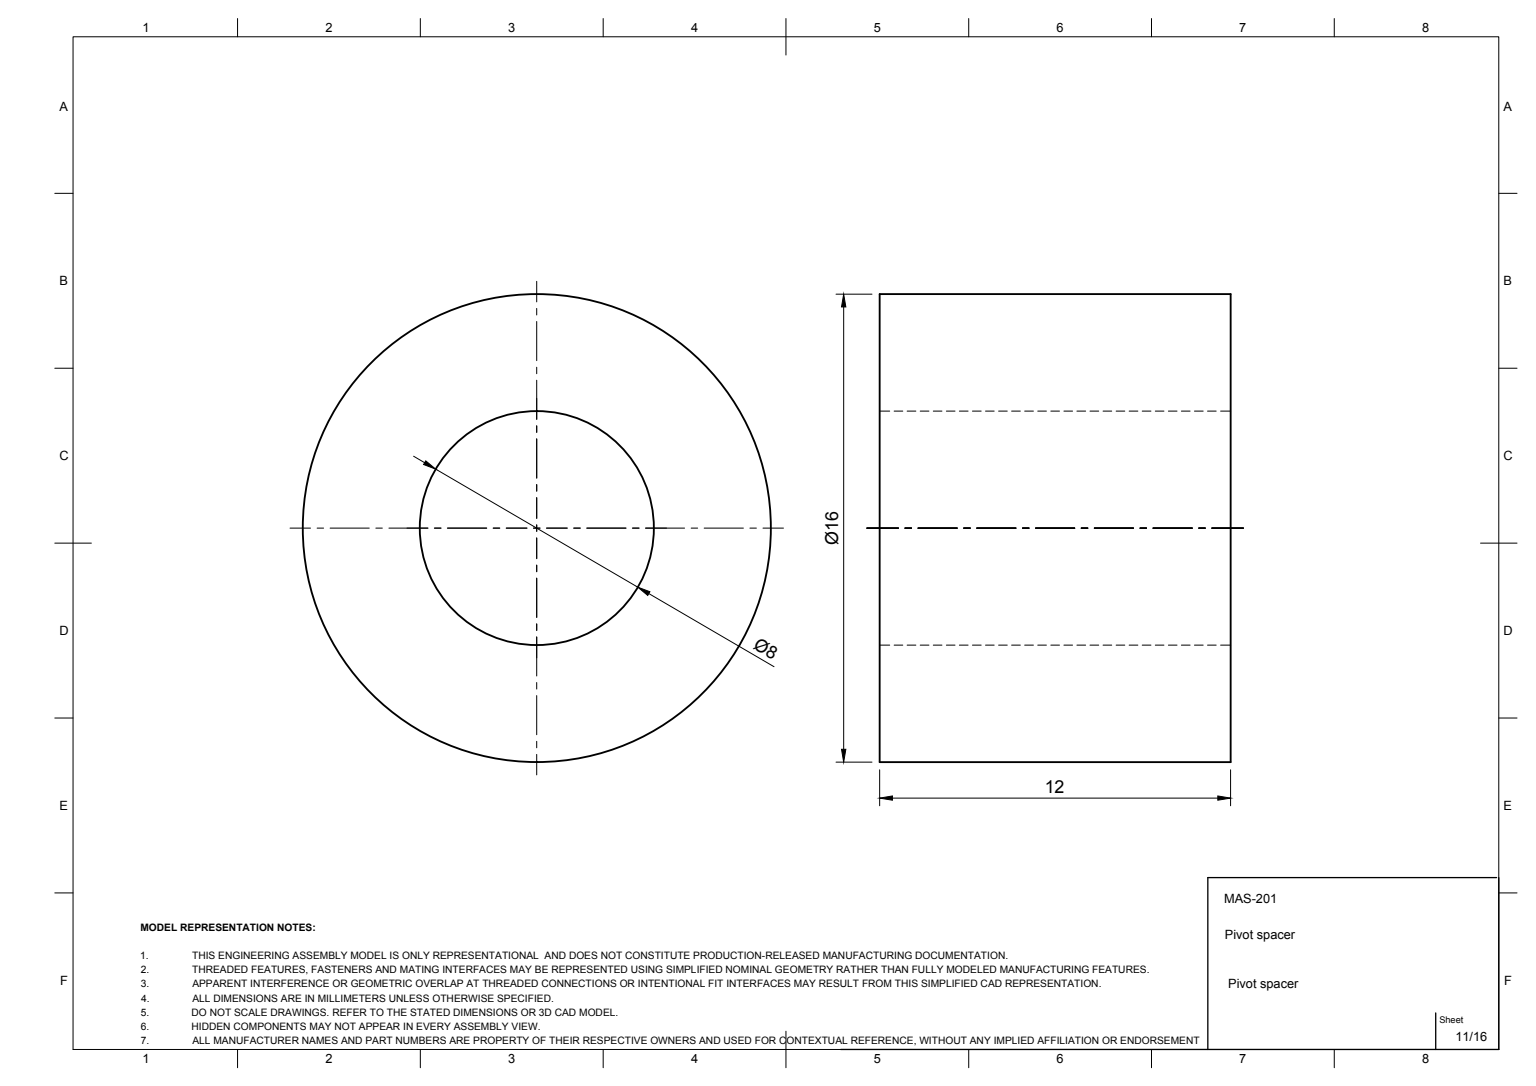
ISO-10303-21;
HEADER;
/* Generated by software containing ST-Developer
 * from STEP Tools, Inc. (www.steptools.com) 
 */

FILE_DESCRIPTION(
/* description */ ('Independent manual two-gate roller-track escapement for nominal30mm d
iameter20mm wide feed rollers. Opposed gates are driven by native capt
ured pin-slot loops with positive curved-slot travel stops at\X\B116de
g. Repeated gate/pin/washer/clip instances, adapted native common bear
ing families, full retaining lips and rotating polymer grip. External 
workpieces, gravity feeder/incline and mount anchors outside assembly.
 No powered-feed compatibility, impact, capacity, safety, force, wear 
or life rating.'),
/* implementation_level */ '2;1');

FILE_NAME(
/* name */ 'Pivot spacer.step',
/* time_stamp */ '2026-11-08T18:43:23-08:00',
/* author */ (''),
/* organization */ (''),
/* preprocessor_version */ 'ST-DEVELOPER v20.2',
/* originating_system */ 'Autodesk Translation Framework v15.17.0.0',
/* authorisation */ '');

FILE_SCHEMA (('AUTOMOTIVE_DESIGN { 1 0 10303 214 3 1 1 }'));
ENDSEC;

DATA;
#10=MECHANICAL_DESIGN_GEOMETRIC_PRESENTATION_REPRESENTATION('',(#465),#19863);
#427=SHAPE_REPRESENTATION_RELATIONSHIP('SRR','None',#19945,#446);
#446=ADVANCED_BREP_SHAPE_REPRESENTATION('',(#484),#19854);
#465=STYLED_ITEM('',(#20042),#484);
#484=MANIFOLD_SOLID_BREP('Body1',#6434);
#848=LINE('',#15905,#1313);
#849=LINE('',#15911,#1314);
#1313=VECTOR('',#8246,4.);
#1314=VECTOR('',#8253,8.);
#1552=CYLINDRICAL_SURFACE('',#7001,4.);
#1553=CYLINDRICAL_SURFACE('',#7004,8.);
#1671=FACE_BOUND('',#2349,.T.);
#1672=FACE_BOUND('',#2351,.T.);
#1933=FACE_OUTER_BOUND('',#2346,.T.);
#1934=FACE_OUTER_BOUND('',#2347,.T.);
#1935=FACE_OUTER_BOUND('',#2348,.T.);
#1936=FACE_OUTER_BOUND('',#2350,.T.);
#2346=EDGE_LOOP('',(#5397,#5398,#5399,#5400));
#2347=EDGE_LOOP('',(#5401,#5402,#5403,#5404));
#2348=EDGE_LOOP('',(#5405));
#2349=EDGE_LOOP('',(#5406));
#2350=EDGE_LOOP('',(#5407));
#2351=EDGE_LOOP('',(#5408));
#2570=CIRCLE('',#7002,4.);
#2571=CIRCLE('',#7003,4.);
#2572=CIRCLE('',#7005,8.);
#2573=CIRCLE('',#7006,8.);
#3044=VERTEX_POINT('',#15902);
#3045=VERTEX_POINT('',#15904);
#3046=VERTEX_POINT('',#15908);
#3047=VERTEX_POINT('',#15910);
#3857=EDGE_CURVE('',#3044,#3044,#2570,.T.);
#3858=EDGE_CURVE('',#3044,#3045,#848,.T.);
#3859=EDGE_CURVE('',#3045,#3045,#2571,.T.);
#3860=EDGE_CURVE('',#3046,#3046,#2572,.T.);
#3861=EDGE_CURVE('',#3046,#3047,#849,.T.);
#3862=EDGE_CURVE('',#3047,#3047,#2573,.T.);
#5397=ORIENTED_EDGE('',*,*,#3857,.F.);
#5398=ORIENTED_EDGE('',*,*,#3858,.T.);
#5399=ORIENTED_EDGE('',*,*,#3859,.T.);
#5400=ORIENTED_EDGE('',*,*,#3858,.F.);
#5401=ORIENTED_EDGE('',*,*,#3860,.F.);
#5402=ORIENTED_EDGE('',*,*,#3861,.T.);
#5403=ORIENTED_EDGE('',*,*,#3862,.T.);
#5404=ORIENTED_EDGE('',*,*,#3861,.F.);
#5405=ORIENTED_EDGE('',*,*,#3860,.T.);
#5406=ORIENTED_EDGE('',*,*,#3857,.T.);
#5407=ORIENTED_EDGE('',*,*,#3862,.F.);
#5408=ORIENTED_EDGE('',*,*,#3859,.F.);
#6024=PLANE('',#7007);
#6025=PLANE('',#7008);
#6312=ADVANCED_FACE('',(#1933),#1552,.F.);
#6313=ADVANCED_FACE('',(#1934),#1553,.T.);
#6314=ADVANCED_FACE('',(#1935,#1671),#6024,.T.);
#6315=ADVANCED_FACE('',(#1936,#1672),#6025,.F.);
#6434=CLOSED_SHELL('',(#6312,#6313,#6314,#6315));
#7000=AXIS2_PLACEMENT_3D('',#15900,#8240,#8241);
#7001=AXIS2_PLACEMENT_3D('',#15901,#8242,#8243);
#7002=AXIS2_PLACEMENT_3D('',#15903,#8244,#8245);
#7003=AXIS2_PLACEMENT_3D('',#15906,#8247,#8248);
#7004=AXIS2_PLACEMENT_3D('',#15907,#8249,#8250);
#7005=AXIS2_PLACEMENT_3D('',#15909,#8251,#8252);
#7006=AXIS2_PLACEMENT_3D('',#15912,#8254,#8255);
#7007=AXIS2_PLACEMENT_3D('',#15913,#8256,#8257);
#7008=AXIS2_PLACEMENT_3D('',#15914,#8258,#8259);
#8240=DIRECTION('axis',(0.,0.,1.));
#8241=DIRECTION('refdir',(1.,0.,0.));
#8242=DIRECTION('center_axis',(0.,0.,1.));
#8243=DIRECTION('ref_axis',(1.,0.,0.));
#8244=DIRECTION('center_axis',(0.,0.,-1.));
#8245=DIRECTION('ref_axis',(1.,0.,0.));
#8246=DIRECTION('',(0.,0.,-1.));
#8247=DIRECTION('center_axis',(0.,0.,-1.));
#8248=DIRECTION('ref_axis',(1.,0.,0.));
#8249=DIRECTION('center_axis',(0.,0.,1.));
#8250=DIRECTION('ref_axis',(1.,0.,0.));
#8251=DIRECTION('center_axis',(0.,0.,1.));
#8252=DIRECTION('ref_axis',(1.,0.,0.));
#8253=DIRECTION('',(0.,0.,-1.));
#8254=DIRECTION('center_axis',(0.,0.,1.));
#8255=DIRECTION('ref_axis',(1.,0.,0.));
#8256=DIRECTION('center_axis',(0.,0.,1.));
#8257=DIRECTION('ref_axis',(1.,0.,0.));
#8258=DIRECTION('center_axis',(0.,0.,1.));
#8259=DIRECTION('ref_axis',(1.,0.,0.));
#15900=CARTESIAN_POINT('',(0.,0.,0.));
#15901=CARTESIAN_POINT('Origin',(0.,0.,0.));
#15902=CARTESIAN_POINT('',(-4.,-4.89858719658941E-16,12.));
#15903=CARTESIAN_POINT('Origin',(0.,0.,12.));
#15904=CARTESIAN_POINT('',(-4.,-4.89858719658941E-16,0.));
#15905=CARTESIAN_POINT('',(-4.,-4.89858719658941E-16,0.));
#15906=CARTESIAN_POINT('Origin',(0.,0.,0.));
#15907=CARTESIAN_POINT('Origin',(0.,0.,0.));
#15908=CARTESIAN_POINT('',(-8.,-9.79717439317883E-16,12.));
#15909=CARTESIAN_POINT('Origin',(0.,0.,12.));
#15910=CARTESIAN_POINT('',(-8.,-9.79717439317883E-16,0.));
#15911=CARTESIAN_POINT('',(-8.,-9.79717439317883E-16,0.));
#15912=CARTESIAN_POINT('Origin',(0.,0.,0.));
#15913=CARTESIAN_POINT('Origin',(0.,0.,12.));
#15914=CARTESIAN_POINT('Origin',(0.,0.,0.));
#19833=UNCERTAINTY_MEASURE_WITH_UNIT(LENGTH_MEASURE(0.01),#19864,
'DISTANCE_ACCURACY_VALUE',
'Maximum model space distance between geometric entities at asserted c
onnectivities');
#19842=UNCERTAINTY_MEASURE_WITH_UNIT(LENGTH_MEASURE(0.01),#19864,
'DISTANCE_ACCURACY_VALUE',
'Maximum model space distance between geometric entities at asserted c
onnectivities');
#19854=(
GEOMETRIC_REPRESENTATION_CONTEXT(3)
GLOBAL_UNCERTAINTY_ASSIGNED_CONTEXT((#19833))
GLOBAL_UNIT_ASSIGNED_CONTEXT((#19864,#19866,#19867))
REPRESENTATION_CONTEXT('','3D')
);
#19863=(
GEOMETRIC_REPRESENTATION_CONTEXT(3)
GLOBAL_UNCERTAINTY_ASSIGNED_CONTEXT((#19842))
GLOBAL_UNIT_ASSIGNED_CONTEXT((#19864,#19866,#19867))
REPRESENTATION_CONTEXT('','3D')
);
#19864=(
LENGTH_UNIT()
NAMED_UNIT(*)
SI_UNIT(.MILLI.,.METRE.)
);
#19866=(
NAMED_UNIT(*)
PLANE_ANGLE_UNIT()
SI_UNIT($,.RADIAN.)
);
#19867=(
NAMED_UNIT(*)
SI_UNIT($,.STERADIAN.)
SOLID_ANGLE_UNIT()
);
#19879=SHAPE_DEFINITION_REPRESENTATION(#19899,#19945);
#19899=PRODUCT_DEFINITION_SHAPE('',$,#19966);
#19945=SHAPE_REPRESENTATION('',(#7000),#19854);
#19954=PRODUCT_DEFINITION_CONTEXT('part definition',#20016,'design');
#19966=PRODUCT_DEFINITION('Pivot spacer','Pivot spacer',#19986,#19954);
#19986=PRODUCT_DEFINITION_FORMATION('',$,#20029);
#20016=APPLICATION_CONTEXT(
'Core Data for Automotive Mechanical Design Process');
#20017=PRODUCT_CONTEXT('part definition',#20016,'mechanical');
#20029=PRODUCT('Pivot spacer','Pivot spacer',$,(#20017));
#20042=PRESENTATION_STYLE_ASSIGNMENT((#20049));
#20049=SURFACE_STYLE_USAGE(.BOTH.,#20056);
#20056=SURFACE_SIDE_STYLE('',(#20063));
#20063=SURFACE_STYLE_FILL_AREA(#20070);
#20070=FILL_AREA_STYLE('Gray',(#20077));
#20077=FILL_AREA_STYLE_COLOUR('Gray',#20084);
#20084=COLOUR_RGB('Gray',0.407843137254902,0.447058823529412,0.498039215686275);
ENDSEC;
END-ISO-10303-21;
